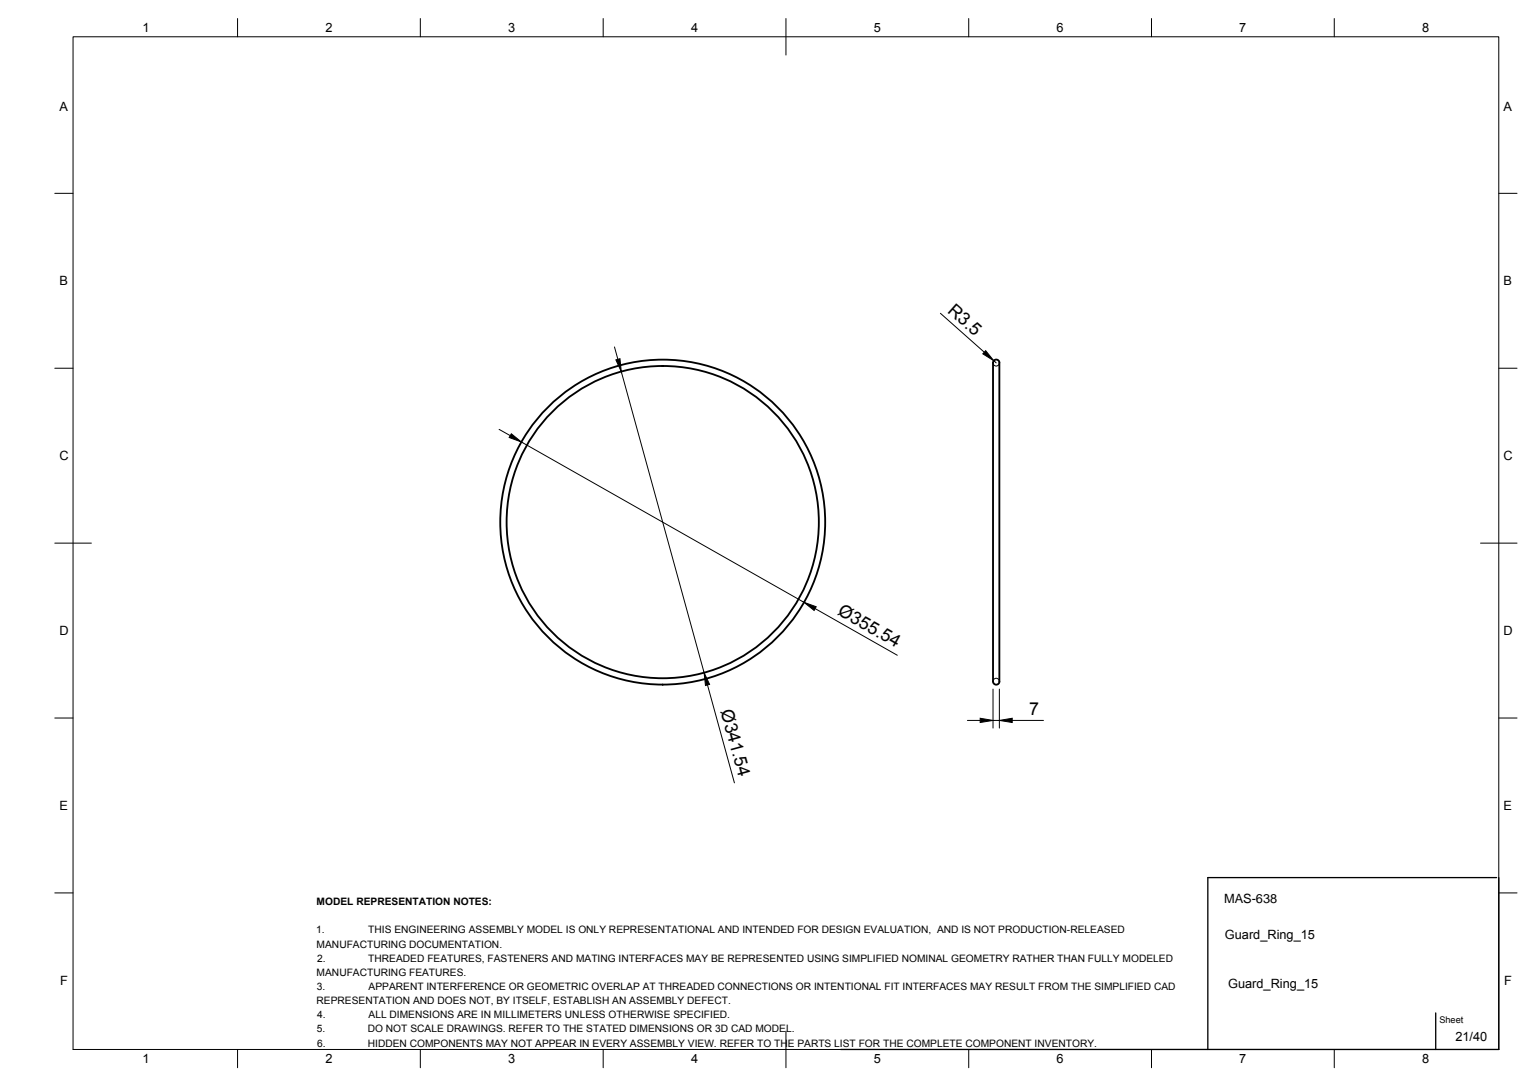
ISO-10303-21;
HEADER;
FILE_DESCRIPTION((''),'2;1');
FILE_NAME('Guard_Ring_15.step','2026-10-09T12:00:21-07:00',(''),(''),'','','');
FILE_SCHEMA (('AUTOMOTIVE_DESIGN { 1 0 10303 214 3 1 1 }'));
ENDSEC;
DATA;
#10=MECHANICAL_DESIGN_GEOMETRIC_PRESENTATION_REPRESENTATION('',(#419),#10334);
#348=SHAPE_REPRESENTATION_RELATIONSHIP('SRR','None',#10464,#380) ;
#380=ADVANCED_BREP_SHAPE_REPRESENTATION('',(#452),#10316) ;
#419=STYLED_ITEM('',(#10631),#452) ;
#452=MANIFOLD_SOLID_BREP('Body1',#3574) ;
#873=FACE_OUTER_BOUND('',#1073,.T.) ;
#1073=EDGE_LOOP('',(#2405,#2406,#2407,#2408)) ;
#1304=CIRCLE('',#4031,0.349999999999999) ;
#1305=CIRCLE('',#4032,17.0768144613668) ;
#1527=VERTEX_POINT('',#5723) ;
#1859=EDGE_CURVE('',#1527,#1527,#1304,.T.) ;
#1860=EDGE_CURVE('',#1527,#1527,#1305,.T.) ;
#2405=ORIENTED_EDGE('',*,*,#1859,.F.) ;
#2406=ORIENTED_EDGE('',*,*,#1860,.T.) ;
#2407=ORIENTED_EDGE('',*,*,#1859,.T.) ;
#2408=ORIENTED_EDGE('',*,*,#1860,.F.) ;
#3319=TOROIDAL_SURFACE('',#4030,17.4268144613668,0.349999999999999) ;
#3381=ADVANCED_FACE('',(#873),#3319,.T.) ;
#3574=CLOSED_SHELL('',(#3381)) ;
#4029=AXIS2_PLACEMENT_3D('',#5721,#4619,#4620) ;
#4030=AXIS2_PLACEMENT_3D('',#5722,#4621,#4622) ;
#4031=AXIS2_PLACEMENT_3D('',#5724,#4623,#4624) ;
#4032=AXIS2_PLACEMENT_3D('',#5725,#4625,#4626) ;
#4619=DIRECTION('axis',(0.,0.,1.)) ;
#4620=DIRECTION('refdir',(1.,0.,0.)) ;
#4621=DIRECTION('center_axis',(-6.42891162084177E-17,-1.,-1.01883556321148E-16)) ;
#4622=DIRECTION('ref_axis',(1.,0.,0.)) ;
#4623=DIRECTION('center_axis',(0.,1.01883556321148E-16,-1.)) ;
#4624=DIRECTION('ref_axis',(-1.,0.,0.)) ;
#4625=DIRECTION('center_axis',(6.42891162084177E-17,1.,1.01883556321148E-16)) ;
#4626=DIRECTION('ref_axis',(1.,-6.42891162084177E-17,-6.55000379205715E-33)) ;
#5721=CARTESIAN_POINT('',(0.,0.,0.)) ;
#5722=CARTESIAN_POINT('Origin',(23.47768801576,67.3831179463143,68.2224337400009)) ;
#5723=CARTESIAN_POINT('',(6.4008735543932,67.3831179463143,68.2224337400009)) ;
#5724=CARTESIAN_POINT('Origin',(6.0508735543932,67.3831179463143,68.2224337400009)) ;
#5725=CARTESIAN_POINT('Origin',(23.47768801576,67.3831179463143,68.2224337400009)) ;
#10279=UNCERTAINTY_MEASURE_WITH_UNIT(LENGTH_MEASURE(0.001),#10335,
'DISTANCE_ACCURACY_VALUE',
'Maximum model space distance between geometric entities at asserted c
onnectivities') ;
#10297=UNCERTAINTY_MEASURE_WITH_UNIT(LENGTH_MEASURE(0.001),#10335,
'DISTANCE_ACCURACY_VALUE',
'Maximum model space distance between geometric entities at asserted c
onnectivities') ;
#10316=(
GEOMETRIC_REPRESENTATION_CONTEXT(3)
GLOBAL_UNCERTAINTY_ASSIGNED_CONTEXT((#10279))
GLOBAL_UNIT_ASSIGNED_CONTEXT((#10335,#10337,#10338))
REPRESENTATION_CONTEXT('','3D')
) ;
#10334=(
GEOMETRIC_REPRESENTATION_CONTEXT(3)
GLOBAL_UNCERTAINTY_ASSIGNED_CONTEXT((#10297))
GLOBAL_UNIT_ASSIGNED_CONTEXT((#10335,#10337,#10338))
REPRESENTATION_CONTEXT('','3D')
) ;
#10335=(
LENGTH_UNIT()
NAMED_UNIT(*)
SI_UNIT(.CENTI.,.METRE.)
) ;
#10337=(
NAMED_UNIT(*)
PLANE_ANGLE_UNIT()
SI_UNIT($,.RADIAN.)
) ;
#10338=(
NAMED_UNIT(*)
SI_UNIT($,.STERADIAN.)
SOLID_ANGLE_UNIT()
) ;
#10357=SHAPE_DEFINITION_REPRESENTATION(#10393,#10464) ;
#10393=PRODUCT_DEFINITION_SHAPE('',$,#10501) ;
#10464=SHAPE_REPRESENTATION('',(#4029),#10316) ;
#10482=PRODUCT_DEFINITION_CONTEXT('part definition',#10592,'design') ;
#10501=PRODUCT_DEFINITION('Guard_Ring_15','Guard_Ring_15',#10537,#10482) ;
#10537=PRODUCT_DEFINITION_FORMATION('',$,#10612) ;
#10592=APPLICATION_CONTEXT(
'Core Data for Automotive Mechanical Design Process') ;
#10593=PRODUCT_CONTEXT('part definition',#10592,'mechanical') ;
#10612=PRODUCT('Guard_Ring_15','Guard_Ring_15',$,(#10593)) ;
#10631=PRESENTATION_STYLE_ASSIGNMENT((#10635)) ;
#10635=SURFACE_STYLE_USAGE(.BOTH.,#10639) ;
#10639=SURFACE_SIDE_STYLE('',(#10643)) ;
#10643=SURFACE_STYLE_FILL_AREA(#10647) ;
#10647=FILL_AREA_STYLE('Opaque(25,25,25)',(#10651)) ;
#10651=FILL_AREA_STYLE_COLOUR('Opaque(25,25,25)',#10655) ;
#10655=COLOUR_RGB('Opaque(25,25,25)', 0.09019608, 0.27058824, 0.51372549) ;
ENDSEC;
END-ISO-10303-21;
